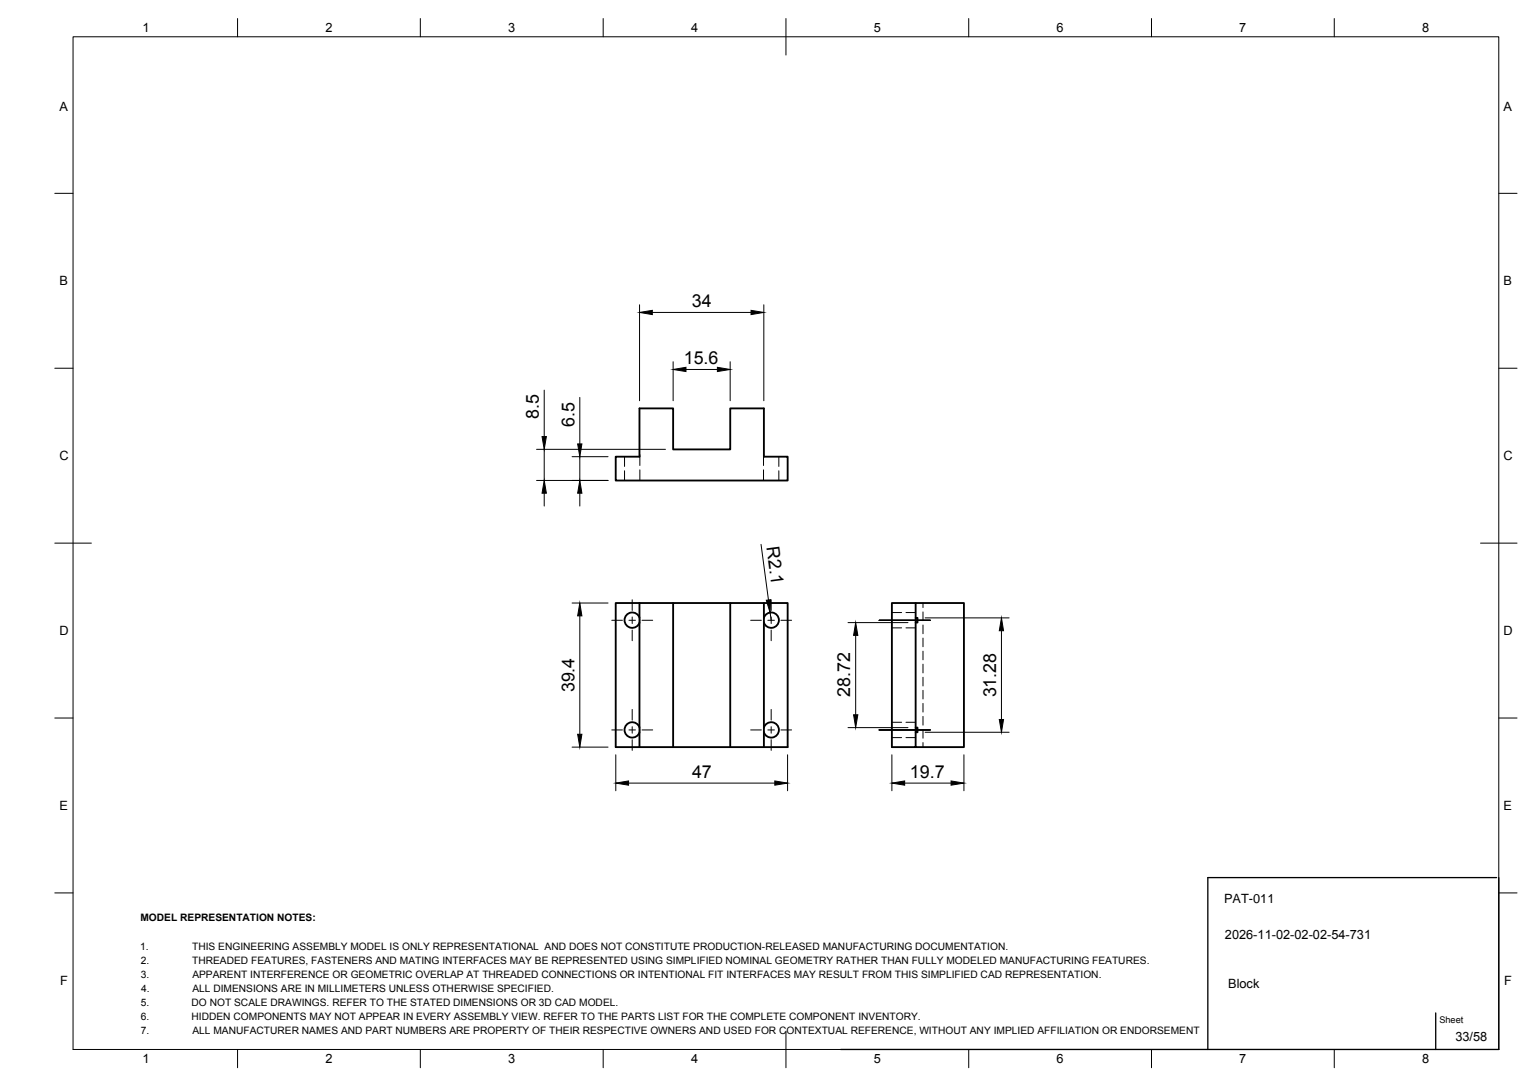
ISO-10303-21;
HEADER;
/* Generated by software containing ST-Developer
 * from STEP Tools, Inc. (www.steptools.com) 
 */

FILE_DESCRIPTION(
/* description */ ('Belt tension measurement rig'),
/* implementation_level */ '2;1');

FILE_NAME(
/* name */ 'Block.step',
/* time_stamp */ '2026-10-28T03:24:44-07:00',
/* author */ (''),
/* organization */ (''),
/* preprocessor_version */ 'ST-DEVELOPER v20.2',
/* originating_system */ 'Autodesk Translation Framework v15.17.0.0',
/* authorisation */ '');

FILE_SCHEMA (('AUTOMOTIVE_DESIGN { 1 0 10303 214 3 1 1 }'));
ENDSEC;

DATA;
#10=MECHANICAL_DESIGN_GEOMETRIC_PRESENTATION_REPRESENTATION('',(#727),#23587);
#609=SHAPE_REPRESENTATION_RELATIONSHIP('SRR','None',#23857,#664);
#664=ADVANCED_BREP_SHAPE_REPRESENTATION('',(#797),#23555);
#727=STYLED_ITEM('',(#24190),#797);
#797=MANIFOLD_SOLID_BREP('Body1',#12232);
#969=FACE_BOUND('',#2535,.T.);
#970=FACE_BOUND('',#2536,.T.);
#971=FACE_BOUND('',#2537,.T.);
#972=FACE_BOUND('',#2538,.T.);
#1201=PLANE('',#13566);
#1202=PLANE('',#13572);
#1203=PLANE('',#13578);
#1204=PLANE('',#13584);
#1205=PLANE('',#13590);
#1206=PLANE('',#13591);
#1207=PLANE('',#13592);
#1208=PLANE('',#13593);
#1209=PLANE('',#13594);
#1210=PLANE('',#13595);
#1211=PLANE('',#13596);
#1212=PLANE('',#13597);
#1213=PLANE('',#13598);
#1214=PLANE('',#13599);
#1215=PLANE('',#13600);
#1216=PLANE('',#13601);
#1217=PLANE('',#13602);
#1218=PLANE('',#13603);
#1677=FACE_OUTER_BOUND('',#2521,.T.);
#1678=FACE_OUTER_BOUND('',#2522,.T.);
#1679=FACE_OUTER_BOUND('',#2523,.T.);
#1680=FACE_OUTER_BOUND('',#2524,.T.);
#1681=FACE_OUTER_BOUND('',#2525,.T.);
#1682=FACE_OUTER_BOUND('',#2526,.T.);
#1683=FACE_OUTER_BOUND('',#2527,.T.);
#1684=FACE_OUTER_BOUND('',#2528,.T.);
#1685=FACE_OUTER_BOUND('',#2529,.T.);
#1686=FACE_OUTER_BOUND('',#2530,.T.);
#1687=FACE_OUTER_BOUND('',#2531,.T.);
#1688=FACE_OUTER_BOUND('',#2532,.T.);
#1689=FACE_OUTER_BOUND('',#2533,.T.);
#1690=FACE_OUTER_BOUND('',#2534,.T.);
#1691=FACE_OUTER_BOUND('',#2539,.T.);
#1692=FACE_OUTER_BOUND('',#2540,.T.);
#1693=FACE_OUTER_BOUND('',#2541,.T.);
#1694=FACE_OUTER_BOUND('',#2542,.T.);
#1695=FACE_OUTER_BOUND('',#2543,.T.);
#1696=FACE_OUTER_BOUND('',#2544,.T.);
#1697=FACE_OUTER_BOUND('',#2545,.T.);
#1698=FACE_OUTER_BOUND('',#2546,.T.);
#2521=EDGE_LOOP('',(#9362,#9363));
#2522=EDGE_LOOP('',(#9364,#9365,#9366,#9367,#9368,#9369,#9370,#9371));
#2523=EDGE_LOOP('',(#9372,#9373));
#2524=EDGE_LOOP('',(#9374,#9375,#9376,#9377,#9378,#9379,#9380,#9381));
#2525=EDGE_LOOP('',(#9382,#9383));
#2526=EDGE_LOOP('',(#9384,#9385,#9386,#9387,#9388,#9389,#9390,#9391));
#2527=EDGE_LOOP('',(#9392,#9393));
#2528=EDGE_LOOP('',(#9394,#9395,#9396,#9397,#9398,#9399,#9400,#9401));
#2529=EDGE_LOOP('',(#9402,#9403,#9404,#9405,#9406,#9407,#9408,#9409,#9410,
#9411,#9412,#9413));
#2530=EDGE_LOOP('',(#9414,#9415,#9416,#9417,#9418,#9419,#9420,#9421,#9422,
#9423,#9424,#9425));
#2531=EDGE_LOOP('',(#9426,#9427,#9428,#9429,#9430,#9431,#9432,#9433,#9434,
#9435,#9436,#9437));
#2532=EDGE_LOOP('',(#9438,#9439,#9440,#9441,#9442,#9443,#9444,#9445,#9446,
#9447));
#2533=EDGE_LOOP('',(#9448,#9449,#9450,#9451));
#2534=EDGE_LOOP('',(#9452,#9453,#9454,#9455));
#2535=EDGE_LOOP('',(#9456));
#2536=EDGE_LOOP('',(#9457));
#2537=EDGE_LOOP('',(#9458));
#2538=EDGE_LOOP('',(#9459));
#2539=EDGE_LOOP('',(#9460,#9461,#9462,#9463));
#2540=EDGE_LOOP('',(#9464,#9465,#9466,#9467,#9468,#9469,#9470,#9471,#9472,
#9473));
#2541=EDGE_LOOP('',(#9474,#9475,#9476,#9477));
#2542=EDGE_LOOP('',(#9478,#9479,#9480,#9481));
#2543=EDGE_LOOP('',(#9482,#9483,#9484,#9485));
#2544=EDGE_LOOP('',(#9486,#9487,#9488,#9489));
#2545=EDGE_LOOP('',(#9490,#9491,#9492,#9493));
#2546=EDGE_LOOP('',(#9494,#9495,#9496,#9497,#9498,#9499,#9500,#9501,#9502,
#9503,#9504,#9505));
#3327=LINE('',#20539,#4078);
#3328=LINE('',#20543,#4079);
#3329=LINE('',#20547,#4080);
#3330=LINE('',#20551,#4081);
#3331=LINE('',#20555,#4082);
#3332=LINE('',#20559,#4083);
#3333=LINE('',#20563,#4084);
#3334=LINE('',#20567,#4085);
#3335=LINE('',#20571,#4086);
#3336=LINE('',#20575,#4087);
#3337=LINE('',#20579,#4088);
#3338=LINE('',#20583,#4089);
#3339=LINE('',#20587,#4090);
#3340=LINE('',#20591,#4091);
#3341=LINE('',#20595,#4092);
#3342=LINE('',#20599,#4093);
#3343=LINE('',#20601,#4094);
#3344=LINE('',#20603,#4095);
#3345=LINE('',#20605,#4096);
#3346=LINE('',#20607,#4097);
#3347=LINE('',#20609,#4098);
#3348=LINE('',#20610,#4099);
#3349=LINE('',#20612,#4100);
#3350=LINE('',#20614,#4101);
#3351=LINE('',#20616,#4102);
#3352=LINE('',#20618,#4103);
#3353=LINE('',#20620,#4104);
#3354=LINE('',#20621,#4105);
#3355=LINE('',#20624,#4106);
#3356=LINE('',#20626,#4107);
#3357=LINE('',#20628,#4108);
#3358=LINE('',#20630,#4109);
#3359=LINE('',#20631,#4110);
#3360=LINE('',#20633,#4111);
#3361=LINE('',#20635,#4112);
#3362=LINE('',#20637,#4113);
#3363=LINE('',#20639,#4114);
#3364=LINE('',#20640,#4115);
#3365=LINE('',#20643,#4116);
#3366=LINE('',#20644,#4117);
#3367=LINE('',#20647,#4118);
#3368=LINE('',#20648,#4119);
#3369=LINE('',#20651,#4120);
#3370=LINE('',#20652,#4121);
#3371=LINE('',#20655,#4122);
#3372=LINE('',#20656,#4123);
#3373=LINE('',#20658,#4124);
#3374=LINE('',#20661,#4125);
#3375=LINE('',#20662,#4126);
#3376=LINE('',#20665,#4127);
#3377=LINE('',#20666,#4128);
#3378=LINE('',#20669,#4129);
#3379=LINE('',#20670,#4130);
#3380=LINE('',#20673,#4131);
#3381=LINE('',#20674,#4132);
#3382=LINE('',#20676,#4133);
#4078=VECTOR('',#16258,1.);
#4079=VECTOR('',#16263,1.);
#4080=VECTOR('',#16266,0.21);
#4081=VECTOR('',#16271,1.);
#4082=VECTOR('',#16274,1.);
#4083=VECTOR('',#16279,1.);
#4084=VECTOR('',#16282,0.21);
#4085=VECTOR('',#16287,1.);
#4086=VECTOR('',#16290,1.);
#4087=VECTOR('',#16295,1.);
#4088=VECTOR('',#16298,0.21);
#4089=VECTOR('',#16303,1.);
#4090=VECTOR('',#16306,1.);
#4091=VECTOR('',#16311,1.);
#4092=VECTOR('',#16314,0.21);
#4093=VECTOR('',#16319,1.);
#4094=VECTOR('',#16322,1.);
#4095=VECTOR('',#16323,1.);
#4096=VECTOR('',#16324,1.);
#4097=VECTOR('',#16325,1.);
#4098=VECTOR('',#16326,1.);
#4099=VECTOR('',#16327,1.);
#4100=VECTOR('',#16330,1.);
#4101=VECTOR('',#16331,1.);
#4102=VECTOR('',#16332,1.);
#4103=VECTOR('',#16333,1.);
#4104=VECTOR('',#16334,1.);
#4105=VECTOR('',#16335,1.);
#4106=VECTOR('',#16338,1.);
#4107=VECTOR('',#16339,1.);
#4108=VECTOR('',#16340,1.);
#4109=VECTOR('',#16341,1.);
#4110=VECTOR('',#16342,1.);
#4111=VECTOR('',#16343,1.);
#4112=VECTOR('',#16344,1.);
#4113=VECTOR('',#16345,1.);
#4114=VECTOR('',#16346,1.);
#4115=VECTOR('',#16347,1.);
#4116=VECTOR('',#16350,1.);
#4117=VECTOR('',#16351,1.);
#4118=VECTOR('',#16354,1.);
#4119=VECTOR('',#16355,1.);
#4120=VECTOR('',#16358,1.);
#4121=VECTOR('',#16359,1.);
#4122=VECTOR('',#16362,1.);
#4123=VECTOR('',#16363,1.);
#4124=VECTOR('',#16366,1.);
#4125=VECTOR('',#16369,1.);
#4126=VECTOR('',#16370,1.);
#4127=VECTOR('',#16373,1.);
#4128=VECTOR('',#16374,1.);
#4129=VECTOR('',#16377,1.);
#4130=VECTOR('',#16378,1.);
#4131=VECTOR('',#16381,1.);
#4132=VECTOR('',#16382,1.);
#4133=VECTOR('',#16385,1.);
#4797=CIRCLE('',#13567,0.21);
#4798=CIRCLE('',#13569,0.21);
#4799=CIRCLE('',#13570,0.21);
#4800=CIRCLE('',#13571,0.21);
#4801=CIRCLE('',#13573,0.21);
#4802=CIRCLE('',#13575,0.21);
#4803=CIRCLE('',#13576,0.21);
#4804=CIRCLE('',#13577,0.21);
#4805=CIRCLE('',#13579,0.21);
#4806=CIRCLE('',#13581,0.21);
#4807=CIRCLE('',#13582,0.21);
#4808=CIRCLE('',#13583,0.21);
#4809=CIRCLE('',#13585,0.21);
#4810=CIRCLE('',#13587,0.21);
#4811=CIRCLE('',#13588,0.21);
#4812=CIRCLE('',#13589,0.21);
#5719=VERTEX_POINT('',#20537);
#5720=VERTEX_POINT('',#20538);
#5721=VERTEX_POINT('',#20542);
#5722=VERTEX_POINT('',#20544);
#5723=VERTEX_POINT('',#20546);
#5724=VERTEX_POINT('',#20549);
#5725=VERTEX_POINT('',#20553);
#5726=VERTEX_POINT('',#20554);
#5727=VERTEX_POINT('',#20558);
#5728=VERTEX_POINT('',#20560);
#5729=VERTEX_POINT('',#20562);
#5730=VERTEX_POINT('',#20565);
#5731=VERTEX_POINT('',#20569);
#5732=VERTEX_POINT('',#20570);
#5733=VERTEX_POINT('',#20574);
#5734=VERTEX_POINT('',#20576);
#5735=VERTEX_POINT('',#20578);
#5736=VERTEX_POINT('',#20581);
#5737=VERTEX_POINT('',#20585);
#5738=VERTEX_POINT('',#20586);
#5739=VERTEX_POINT('',#20590);
#5740=VERTEX_POINT('',#20592);
#5741=VERTEX_POINT('',#20594);
#5742=VERTEX_POINT('',#20597);
#5743=VERTEX_POINT('',#20602);
#5744=VERTEX_POINT('',#20604);
#5745=VERTEX_POINT('',#20606);
#5746=VERTEX_POINT('',#20608);
#5747=VERTEX_POINT('',#20613);
#5748=VERTEX_POINT('',#20615);
#5749=VERTEX_POINT('',#20617);
#5750=VERTEX_POINT('',#20619);
#5751=VERTEX_POINT('',#20623);
#5752=VERTEX_POINT('',#20625);
#5753=VERTEX_POINT('',#20627);
#5754=VERTEX_POINT('',#20629);
#5755=VERTEX_POINT('',#20632);
#5756=VERTEX_POINT('',#20634);
#5757=VERTEX_POINT('',#20636);
#5758=VERTEX_POINT('',#20638);
#5759=VERTEX_POINT('',#20642);
#5760=VERTEX_POINT('',#20646);
#5761=VERTEX_POINT('',#20650);
#5762=VERTEX_POINT('',#20654);
#5763=VERTEX_POINT('',#20660);
#5764=VERTEX_POINT('',#20664);
#5765=VERTEX_POINT('',#20668);
#5766=VERTEX_POINT('',#20672);
#7040=EDGE_CURVE('',#5719,#5720,#3327,.T.);
#7041=EDGE_CURVE('',#5719,#5720,#4797,.T.);
#7042=EDGE_CURVE('',#5721,#5719,#3328,.T.);
#7043=EDGE_CURVE('',#5722,#5721,#4798,.T.);
#7044=EDGE_CURVE('',#5722,#5723,#3329,.T.);
#7045=EDGE_CURVE('',#5723,#5723,#4799,.T.);
#7046=EDGE_CURVE('',#5724,#5722,#4800,.T.);
#7047=EDGE_CURVE('',#5720,#5724,#3330,.T.);
#7048=EDGE_CURVE('',#5725,#5726,#3331,.T.);
#7049=EDGE_CURVE('',#5725,#5726,#4801,.T.);
#7050=EDGE_CURVE('',#5727,#5725,#3332,.T.);
#7051=EDGE_CURVE('',#5728,#5727,#4802,.T.);
#7052=EDGE_CURVE('',#5728,#5729,#3333,.T.);
#7053=EDGE_CURVE('',#5729,#5729,#4803,.T.);
#7054=EDGE_CURVE('',#5730,#5728,#4804,.T.);
#7055=EDGE_CURVE('',#5726,#5730,#3334,.T.);
#7056=EDGE_CURVE('',#5731,#5732,#3335,.T.);
#7057=EDGE_CURVE('',#5731,#5732,#4805,.T.);
#7058=EDGE_CURVE('',#5733,#5731,#3336,.T.);
#7059=EDGE_CURVE('',#5734,#5733,#4806,.T.);
#7060=EDGE_CURVE('',#5734,#5735,#3337,.T.);
#7061=EDGE_CURVE('',#5735,#5735,#4807,.T.);
#7062=EDGE_CURVE('',#5736,#5734,#4808,.T.);
#7063=EDGE_CURVE('',#5732,#5736,#3338,.T.);
#7064=EDGE_CURVE('',#5737,#5738,#3339,.T.);
#7065=EDGE_CURVE('',#5737,#5738,#4809,.T.);
#7066=EDGE_CURVE('',#5739,#5737,#3340,.T.);
#7067=EDGE_CURVE('',#5740,#5739,#4810,.T.);
#7068=EDGE_CURVE('',#5740,#5741,#3341,.T.);
#7069=EDGE_CURVE('',#5741,#5741,#4811,.T.);
#7070=EDGE_CURVE('',#5742,#5740,#4812,.T.);
#7071=EDGE_CURVE('',#5738,#5742,#3342,.T.);
#7072=EDGE_CURVE('',#5724,#5733,#3343,.T.);
#7073=EDGE_CURVE('',#5736,#5743,#3344,.T.);
#7074=EDGE_CURVE('',#5744,#5743,#3345,.T.);
#7075=EDGE_CURVE('',#5744,#5745,#3346,.T.);
#7076=EDGE_CURVE('',#5746,#5745,#3347,.T.);
#7077=EDGE_CURVE('',#5746,#5721,#3348,.T.);
#7078=EDGE_CURVE('',#5730,#5739,#3349,.T.);
#7079=EDGE_CURVE('',#5742,#5747,#3350,.T.);
#7080=EDGE_CURVE('',#5748,#5747,#3351,.T.);
#7081=EDGE_CURVE('',#5749,#5748,#3352,.T.);
#7082=EDGE_CURVE('',#5750,#5749,#3353,.T.);
#7083=EDGE_CURVE('',#5750,#5727,#3354,.T.);
#7084=EDGE_CURVE('',#5743,#5751,#3355,.T.);
#7085=EDGE_CURVE('',#5751,#5752,#3356,.T.);
#7086=EDGE_CURVE('',#5752,#5753,#3357,.T.);
#7087=EDGE_CURVE('',#5753,#5754,#3358,.T.);
#7088=EDGE_CURVE('',#5754,#5750,#3359,.T.);
#7089=EDGE_CURVE('',#5749,#5755,#3360,.T.);
#7090=EDGE_CURVE('',#5755,#5756,#3361,.T.);
#7091=EDGE_CURVE('',#5756,#5757,#3362,.T.);
#7092=EDGE_CURVE('',#5757,#5758,#3363,.T.);
#7093=EDGE_CURVE('',#5758,#5744,#3364,.T.);
#7094=EDGE_CURVE('',#5759,#5746,#3365,.T.);
#7095=EDGE_CURVE('',#5751,#5759,#3366,.T.);
#7096=EDGE_CURVE('',#5760,#5759,#3367,.T.);
#7097=EDGE_CURVE('',#5752,#5760,#3368,.T.);
#7098=EDGE_CURVE('',#5761,#5760,#3369,.T.);
#7099=EDGE_CURVE('',#5753,#5761,#3370,.T.);
#7100=EDGE_CURVE('',#5762,#5761,#3371,.T.);
#7101=EDGE_CURVE('',#5754,#5762,#3372,.T.);
#7102=EDGE_CURVE('',#5747,#5762,#3373,.T.);
#7103=EDGE_CURVE('',#5763,#5748,#3374,.T.);
#7104=EDGE_CURVE('',#5755,#5763,#3375,.T.);
#7105=EDGE_CURVE('',#5764,#5763,#3376,.T.);
#7106=EDGE_CURVE('',#5756,#5764,#3377,.T.);
#7107=EDGE_CURVE('',#5765,#5764,#3378,.T.);
#7108=EDGE_CURVE('',#5757,#5765,#3379,.T.);
#7109=EDGE_CURVE('',#5766,#5765,#3380,.T.);
#7110=EDGE_CURVE('',#5758,#5766,#3381,.T.);
#7111=EDGE_CURVE('',#5745,#5766,#3382,.T.);
#9362=ORIENTED_EDGE('',*,*,#7040,.F.);
#9363=ORIENTED_EDGE('',*,*,#7041,.T.);
#9364=ORIENTED_EDGE('',*,*,#7042,.F.);
#9365=ORIENTED_EDGE('',*,*,#7043,.F.);
#9366=ORIENTED_EDGE('',*,*,#7044,.T.);
#9367=ORIENTED_EDGE('',*,*,#7045,.F.);
#9368=ORIENTED_EDGE('',*,*,#7044,.F.);
#9369=ORIENTED_EDGE('',*,*,#7046,.F.);
#9370=ORIENTED_EDGE('',*,*,#7047,.F.);
#9371=ORIENTED_EDGE('',*,*,#7041,.F.);
#9372=ORIENTED_EDGE('',*,*,#7048,.F.);
#9373=ORIENTED_EDGE('',*,*,#7049,.T.);
#9374=ORIENTED_EDGE('',*,*,#7050,.F.);
#9375=ORIENTED_EDGE('',*,*,#7051,.F.);
#9376=ORIENTED_EDGE('',*,*,#7052,.T.);
#9377=ORIENTED_EDGE('',*,*,#7053,.F.);
#9378=ORIENTED_EDGE('',*,*,#7052,.F.);
#9379=ORIENTED_EDGE('',*,*,#7054,.F.);
#9380=ORIENTED_EDGE('',*,*,#7055,.F.);
#9381=ORIENTED_EDGE('',*,*,#7049,.F.);
#9382=ORIENTED_EDGE('',*,*,#7056,.F.);
#9383=ORIENTED_EDGE('',*,*,#7057,.T.);
#9384=ORIENTED_EDGE('',*,*,#7058,.F.);
#9385=ORIENTED_EDGE('',*,*,#7059,.F.);
#9386=ORIENTED_EDGE('',*,*,#7060,.T.);
#9387=ORIENTED_EDGE('',*,*,#7061,.F.);
#9388=ORIENTED_EDGE('',*,*,#7060,.F.);
#9389=ORIENTED_EDGE('',*,*,#7062,.F.);
#9390=ORIENTED_EDGE('',*,*,#7063,.F.);
#9391=ORIENTED_EDGE('',*,*,#7057,.F.);
#9392=ORIENTED_EDGE('',*,*,#7064,.F.);
#9393=ORIENTED_EDGE('',*,*,#7065,.T.);
#9394=ORIENTED_EDGE('',*,*,#7066,.F.);
#9395=ORIENTED_EDGE('',*,*,#7067,.F.);
#9396=ORIENTED_EDGE('',*,*,#7068,.T.);
#9397=ORIENTED_EDGE('',*,*,#7069,.F.);
#9398=ORIENTED_EDGE('',*,*,#7068,.F.);
#9399=ORIENTED_EDGE('',*,*,#7070,.F.);
#9400=ORIENTED_EDGE('',*,*,#7071,.F.);
#9401=ORIENTED_EDGE('',*,*,#7065,.F.);
#9402=ORIENTED_EDGE('',*,*,#7042,.T.);
#9403=ORIENTED_EDGE('',*,*,#7040,.T.);
#9404=ORIENTED_EDGE('',*,*,#7047,.T.);
#9405=ORIENTED_EDGE('',*,*,#7072,.T.);
#9406=ORIENTED_EDGE('',*,*,#7058,.T.);
#9407=ORIENTED_EDGE('',*,*,#7056,.T.);
#9408=ORIENTED_EDGE('',*,*,#7063,.T.);
#9409=ORIENTED_EDGE('',*,*,#7073,.T.);
#9410=ORIENTED_EDGE('',*,*,#7074,.F.);
#9411=ORIENTED_EDGE('',*,*,#7075,.T.);
#9412=ORIENTED_EDGE('',*,*,#7076,.F.);
#9413=ORIENTED_EDGE('',*,*,#7077,.T.);
#9414=ORIENTED_EDGE('',*,*,#7050,.T.);
#9415=ORIENTED_EDGE('',*,*,#7048,.T.);
#9416=ORIENTED_EDGE('',*,*,#7055,.T.);
#9417=ORIENTED_EDGE('',*,*,#7078,.T.);
#9418=ORIENTED_EDGE('',*,*,#7066,.T.);
#9419=ORIENTED_EDGE('',*,*,#7064,.T.);
#9420=ORIENTED_EDGE('',*,*,#7071,.T.);
#9421=ORIENTED_EDGE('',*,*,#7079,.T.);
#9422=ORIENTED_EDGE('',*,*,#7080,.F.);
#9423=ORIENTED_EDGE('',*,*,#7081,.F.);
#9424=ORIENTED_EDGE('',*,*,#7082,.F.);
#9425=ORIENTED_EDGE('',*,*,#7083,.T.);
#9426=ORIENTED_EDGE('',*,*,#7074,.T.);
#9427=ORIENTED_EDGE('',*,*,#7084,.T.);
#9428=ORIENTED_EDGE('',*,*,#7085,.T.);
#9429=ORIENTED_EDGE('',*,*,#7086,.T.);
#9430=ORIENTED_EDGE('',*,*,#7087,.T.);
#9431=ORIENTED_EDGE('',*,*,#7088,.T.);
#9432=ORIENTED_EDGE('',*,*,#7082,.T.);
#9433=ORIENTED_EDGE('',*,*,#7089,.T.);
#9434=ORIENTED_EDGE('',*,*,#7090,.T.);
#9435=ORIENTED_EDGE('',*,*,#7091,.T.);
#9436=ORIENTED_EDGE('',*,*,#7092,.T.);
#9437=ORIENTED_EDGE('',*,*,#7093,.T.);
#9438=ORIENTED_EDGE('',*,*,#7046,.T.);
#9439=ORIENTED_EDGE('',*,*,#7043,.T.);
#9440=ORIENTED_EDGE('',*,*,#7077,.F.);
#9441=ORIENTED_EDGE('',*,*,#7094,.F.);
#9442=ORIENTED_EDGE('',*,*,#7095,.F.);
#9443=ORIENTED_EDGE('',*,*,#7084,.F.);
#9444=ORIENTED_EDGE('',*,*,#7073,.F.);
#9445=ORIENTED_EDGE('',*,*,#7062,.T.);
#9446=ORIENTED_EDGE('',*,*,#7059,.T.);
#9447=ORIENTED_EDGE('',*,*,#7072,.F.);
#9448=ORIENTED_EDGE('',*,*,#7095,.T.);
#9449=ORIENTED_EDGE('',*,*,#7096,.F.);
#9450=ORIENTED_EDGE('',*,*,#7097,.F.);
#9451=ORIENTED_EDGE('',*,*,#7085,.F.);
#9452=ORIENTED_EDGE('',*,*,#7097,.T.);
#9453=ORIENTED_EDGE('',*,*,#7098,.F.);
#9454=ORIENTED_EDGE('',*,*,#7099,.F.);
#9455=ORIENTED_EDGE('',*,*,#7086,.F.);
#9456=ORIENTED_EDGE('',*,*,#7045,.T.);
#9457=ORIENTED_EDGE('',*,*,#7053,.T.);
#9458=ORIENTED_EDGE('',*,*,#7061,.T.);
#9459=ORIENTED_EDGE('',*,*,#7069,.T.);
#9460=ORIENTED_EDGE('',*,*,#7099,.T.);
#9461=ORIENTED_EDGE('',*,*,#7100,.F.);
#9462=ORIENTED_EDGE('',*,*,#7101,.F.);
#9463=ORIENTED_EDGE('',*,*,#7087,.F.);
#9464=ORIENTED_EDGE('',*,*,#7054,.T.);
#9465=ORIENTED_EDGE('',*,*,#7051,.T.);
#9466=ORIENTED_EDGE('',*,*,#7083,.F.);
#9467=ORIENTED_EDGE('',*,*,#7088,.F.);
#9468=ORIENTED_EDGE('',*,*,#7101,.T.);
#9469=ORIENTED_EDGE('',*,*,#7102,.F.);
#9470=ORIENTED_EDGE('',*,*,#7079,.F.);
#9471=ORIENTED_EDGE('',*,*,#7070,.T.);
#9472=ORIENTED_EDGE('',*,*,#7067,.T.);
#9473=ORIENTED_EDGE('',*,*,#7078,.F.);
#9474=ORIENTED_EDGE('',*,*,#7081,.T.);
#9475=ORIENTED_EDGE('',*,*,#7103,.F.);
#9476=ORIENTED_EDGE('',*,*,#7104,.F.);
#9477=ORIENTED_EDGE('',*,*,#7089,.F.);
#9478=ORIENTED_EDGE('',*,*,#7104,.T.);
#9479=ORIENTED_EDGE('',*,*,#7105,.F.);
#9480=ORIENTED_EDGE('',*,*,#7106,.F.);
#9481=ORIENTED_EDGE('',*,*,#7090,.F.);
#9482=ORIENTED_EDGE('',*,*,#7106,.T.);
#9483=ORIENTED_EDGE('',*,*,#7107,.F.);
#9484=ORIENTED_EDGE('',*,*,#7108,.F.);
#9485=ORIENTED_EDGE('',*,*,#7091,.F.);
#9486=ORIENTED_EDGE('',*,*,#7108,.T.);
#9487=ORIENTED_EDGE('',*,*,#7109,.F.);
#9488=ORIENTED_EDGE('',*,*,#7110,.F.);
#9489=ORIENTED_EDGE('',*,*,#7092,.F.);
#9490=ORIENTED_EDGE('',*,*,#7110,.T.);
#9491=ORIENTED_EDGE('',*,*,#7111,.F.);
#9492=ORIENTED_EDGE('',*,*,#7075,.F.);
#9493=ORIENTED_EDGE('',*,*,#7093,.F.);
#9494=ORIENTED_EDGE('',*,*,#7076,.T.);
#9495=ORIENTED_EDGE('',*,*,#7111,.T.);
#9496=ORIENTED_EDGE('',*,*,#7109,.T.);
#9497=ORIENTED_EDGE('',*,*,#7107,.T.);
#9498=ORIENTED_EDGE('',*,*,#7105,.T.);
#9499=ORIENTED_EDGE('',*,*,#7103,.T.);
#9500=ORIENTED_EDGE('',*,*,#7080,.T.);
#9501=ORIENTED_EDGE('',*,*,#7102,.T.);
#9502=ORIENTED_EDGE('',*,*,#7100,.T.);
#9503=ORIENTED_EDGE('',*,*,#7098,.T.);
#9504=ORIENTED_EDGE('',*,*,#7096,.T.);
#9505=ORIENTED_EDGE('',*,*,#7094,.T.);
#11297=CYLINDRICAL_SURFACE('',#13568,0.21);
#11298=CYLINDRICAL_SURFACE('',#13574,0.21);
#11299=CYLINDRICAL_SURFACE('',#13580,0.21);
#11300=CYLINDRICAL_SURFACE('',#13586,0.21);
#11818=ADVANCED_FACE('',(#1677),#1201,.T.);
#11819=ADVANCED_FACE('',(#1678),#11297,.F.);
#11820=ADVANCED_FACE('',(#1679),#1202,.T.);
#11821=ADVANCED_FACE('',(#1680),#11298,.F.);
#11822=ADVANCED_FACE('',(#1681),#1203,.T.);
#11823=ADVANCED_FACE('',(#1682),#11299,.F.);
#11824=ADVANCED_FACE('',(#1683),#1204,.T.);
#11825=ADVANCED_FACE('',(#1684),#11300,.F.);
#11826=ADVANCED_FACE('',(#1685),#1205,.T.);
#11827=ADVANCED_FACE('',(#1686),#1206,.T.);
#11828=ADVANCED_FACE('',(#1687),#1207,.T.);
#11829=ADVANCED_FACE('',(#1688),#1208,.T.);
#11830=ADVANCED_FACE('',(#1689),#1209,.T.);
#11831=ADVANCED_FACE('',(#1690,#969,#970,#971,#972),#1210,.T.);
#11832=ADVANCED_FACE('',(#1691),#1211,.T.);
#11833=ADVANCED_FACE('',(#1692),#1212,.T.);
#11834=ADVANCED_FACE('',(#1693),#1213,.T.);
#11835=ADVANCED_FACE('',(#1694),#1214,.T.);
#11836=ADVANCED_FACE('',(#1695),#1215,.T.);
#11837=ADVANCED_FACE('',(#1696),#1216,.T.);
#11838=ADVANCED_FACE('',(#1697),#1217,.T.);
#11839=ADVANCED_FACE('',(#1698),#1218,.T.);
#12232=CLOSED_SHELL('',(#11818,#11819,#11820,#11821,#11822,#11823,#11824,
#11825,#11826,#11827,#11828,#11829,#11830,#11831,#11832,#11833,#11834,#11835,
#11836,#11837,#11838,#11839));
#13565=AXIS2_PLACEMENT_3D('',#20535,#16254,#16255);
#13566=AXIS2_PLACEMENT_3D('',#20536,#16256,#16257);
#13567=AXIS2_PLACEMENT_3D('',#20540,#16259,#16260);
#13568=AXIS2_PLACEMENT_3D('',#20541,#16261,#16262);
#13569=AXIS2_PLACEMENT_3D('',#20545,#16264,#16265);
#13570=AXIS2_PLACEMENT_3D('',#20548,#16267,#16268);
#13571=AXIS2_PLACEMENT_3D('',#20550,#16269,#16270);
#13572=AXIS2_PLACEMENT_3D('',#20552,#16272,#16273);
#13573=AXIS2_PLACEMENT_3D('',#20556,#16275,#16276);
#13574=AXIS2_PLACEMENT_3D('',#20557,#16277,#16278);
#13575=AXIS2_PLACEMENT_3D('',#20561,#16280,#16281);
#13576=AXIS2_PLACEMENT_3D('',#20564,#16283,#16284);
#13577=AXIS2_PLACEMENT_3D('',#20566,#16285,#16286);
#13578=AXIS2_PLACEMENT_3D('',#20568,#16288,#16289);
#13579=AXIS2_PLACEMENT_3D('',#20572,#16291,#16292);
#13580=AXIS2_PLACEMENT_3D('',#20573,#16293,#16294);
#13581=AXIS2_PLACEMENT_3D('',#20577,#16296,#16297);
#13582=AXIS2_PLACEMENT_3D('',#20580,#16299,#16300);
#13583=AXIS2_PLACEMENT_3D('',#20582,#16301,#16302);
#13584=AXIS2_PLACEMENT_3D('',#20584,#16304,#16305);
#13585=AXIS2_PLACEMENT_3D('',#20588,#16307,#16308);
#13586=AXIS2_PLACEMENT_3D('',#20589,#16309,#16310);
#13587=AXIS2_PLACEMENT_3D('',#20593,#16312,#16313);
#13588=AXIS2_PLACEMENT_3D('',#20596,#16315,#16316);
#13589=AXIS2_PLACEMENT_3D('',#20598,#16317,#16318);
#13590=AXIS2_PLACEMENT_3D('',#20600,#16320,#16321);
#13591=AXIS2_PLACEMENT_3D('',#20611,#16328,#16329);
#13592=AXIS2_PLACEMENT_3D('',#20622,#16336,#16337);
#13593=AXIS2_PLACEMENT_3D('',#20641,#16348,#16349);
#13594=AXIS2_PLACEMENT_3D('',#20645,#16352,#16353);
#13595=AXIS2_PLACEMENT_3D('',#20649,#16356,#16357);
#13596=AXIS2_PLACEMENT_3D('',#20653,#16360,#16361);
#13597=AXIS2_PLACEMENT_3D('',#20657,#16364,#16365);
#13598=AXIS2_PLACEMENT_3D('',#20659,#16367,#16368);
#13599=AXIS2_PLACEMENT_3D('',#20663,#16371,#16372);
#13600=AXIS2_PLACEMENT_3D('',#20667,#16375,#16376);
#13601=AXIS2_PLACEMENT_3D('',#20671,#16379,#16380);
#13602=AXIS2_PLACEMENT_3D('',#20675,#16383,#16384);
#13603=AXIS2_PLACEMENT_3D('',#20677,#16386,#16387);
#16254=DIRECTION('axis',(0.,0.,1.));
#16255=DIRECTION('refdir',(1.,0.,0.));
#16256=DIRECTION('center_axis',(0.,0.,1.));
#16257=DIRECTION('ref_axis',(1.,0.,0.));
#16258=DIRECTION('',(-1.,0.,0.));
#16259=DIRECTION('center_axis',(0.,0.,1.));
#16260=DIRECTION('ref_axis',(1.,0.,0.));
#16261=DIRECTION('center_axis',(0.,0.,1.));
#16262=DIRECTION('ref_axis',(1.,0.,0.));
#16263=DIRECTION('',(0.,0.,-1.));
#16264=DIRECTION('center_axis',(0.,0.,1.));
#16265=DIRECTION('ref_axis',(1.,0.,0.));
#16266=DIRECTION('',(0.,0.,1.));
#16267=DIRECTION('center_axis',(0.,0.,-1.));
#16268=DIRECTION('ref_axis',(1.,0.,0.));
#16269=DIRECTION('center_axis',(0.,0.,1.));
#16270=DIRECTION('ref_axis',(1.,0.,0.));
#16271=DIRECTION('',(0.,0.,1.));
#16272=DIRECTION('center_axis',(0.,0.,1.));
#16273=DIRECTION('ref_axis',(1.,0.,0.));
#16274=DIRECTION('',(1.,0.,0.));
#16275=DIRECTION('center_axis',(0.,0.,1.));
#16276=DIRECTION('ref_axis',(1.,0.,0.));
#16277=DIRECTION('center_axis',(0.,0.,1.));
#16278=DIRECTION('ref_axis',(1.,0.,0.));
#16279=DIRECTION('',(0.,0.,-1.));
#16280=DIRECTION('center_axis',(0.,0.,1.));
#16281=DIRECTION('ref_axis',(1.,0.,0.));
#16282=DIRECTION('',(0.,0.,1.));
#16283=DIRECTION('center_axis',(0.,0.,-1.));
#16284=DIRECTION('ref_axis',(1.,0.,0.));
#16285=DIRECTION('center_axis',(0.,0.,1.));
#16286=DIRECTION('ref_axis',(1.,0.,0.));
#16287=DIRECTION('',(0.,0.,1.));
#16288=DIRECTION('center_axis',(0.,0.,1.));
#16289=DIRECTION('ref_axis',(1.,0.,0.));
#16290=DIRECTION('',(-1.,0.,0.));
#16291=DIRECTION('center_axis',(0.,0.,1.));
#16292=DIRECTION('ref_axis',(1.,0.,0.));
#16293=DIRECTION('center_axis',(0.,0.,1.));
#16294=DIRECTION('ref_axis',(1.,0.,0.));
#16295=DIRECTION('',(0.,0.,-1.));
#16296=DIRECTION('center_axis',(0.,0.,1.));
#16297=DIRECTION('ref_axis',(1.,0.,0.));
#16298=DIRECTION('',(0.,0.,1.));
#16299=DIRECTION('center_axis',(0.,0.,-1.));
#16300=DIRECTION('ref_axis',(1.,0.,0.));
#16301=DIRECTION('center_axis',(0.,0.,1.));
#16302=DIRECTION('ref_axis',(1.,0.,0.));
#16303=DIRECTION('',(0.,0.,1.));
#16304=DIRECTION('center_axis',(0.,0.,1.));
#16305=DIRECTION('ref_axis',(1.,0.,0.));
#16306=DIRECTION('',(1.,0.,0.));
#16307=DIRECTION('center_axis',(0.,0.,1.));
#16308=DIRECTION('ref_axis',(1.,0.,0.));
#16309=DIRECTION('center_axis',(0.,0.,1.));
#16310=DIRECTION('ref_axis',(1.,0.,0.));
#16311=DIRECTION('',(0.,0.,-1.));
#16312=DIRECTION('center_axis',(0.,0.,1.));
#16313=DIRECTION('ref_axis',(1.,0.,0.));
#16314=DIRECTION('',(0.,0.,1.));
#16315=DIRECTION('center_axis',(0.,0.,-1.));
#16316=DIRECTION('ref_axis',(1.,0.,0.));
#16317=DIRECTION('center_axis',(0.,0.,1.));
#16318=DIRECTION('ref_axis',(1.,0.,0.));
#16319=DIRECTION('',(0.,0.,1.));
#16320=DIRECTION('center_axis',(0.,-1.,0.));
#16321=DIRECTION('ref_axis',(0.,0.,-1.));
#16322=DIRECTION('',(-1.,0.,0.));
#16323=DIRECTION('',(-1.,0.,0.));
#16324=DIRECTION('',(0.,0.,1.));
#16325=DIRECTION('',(1.,0.,0.));
#16326=DIRECTION('',(0.,0.,-1.));
#16327=DIRECTION('',(-1.,0.,0.));
#16328=DIRECTION('center_axis',(0.,1.,0.));
#16329=DIRECTION('ref_axis',(0.,0.,1.));
#16330=DIRECTION('',(1.,0.,0.));
#16331=DIRECTION('',(1.,0.,0.));
#16332=DIRECTION('',(0.,0.,1.));
#16333=DIRECTION('',(1.,0.,0.));
#16334=DIRECTION('',(0.,0.,-1.));
#16335=DIRECTION('',(1.,0.,0.));
#16336=DIRECTION('center_axis',(-1.,0.,0.));
#16337=DIRECTION('ref_axis',(0.,0.,1.));
#16338=DIRECTION('',(0.,-1.,0.));
#16339=DIRECTION('',(0.,0.,1.));
#16340=DIRECTION('',(0.,1.,0.));
#16341=DIRECTION('',(0.,0.,-1.));
#16342=DIRECTION('',(0.,-1.,0.));
#16343=DIRECTION('',(0.,-1.,0.));
#16344=DIRECTION('',(0.,0.,1.));
#16345=DIRECTION('',(0.,-1.,0.));
#16346=DIRECTION('',(0.,0.,-1.));
#16347=DIRECTION('',(0.,-1.,0.));
#16348=DIRECTION('center_axis',(0.,0.,-1.));
#16349=DIRECTION('ref_axis',(0.,1.,0.));
#16350=DIRECTION('',(0.,1.,0.));
#16351=DIRECTION('',(1.,0.,0.));
#16352=DIRECTION('center_axis',(0.,-1.,0.));
#16353=DIRECTION('ref_axis',(0.,0.,-1.));
#16354=DIRECTION('',(0.,0.,-1.));
#16355=DIRECTION('',(1.,0.,0.));
#16356=DIRECTION('center_axis',(0.,0.,1.));
#16357=DIRECTION('ref_axis',(0.,-1.,0.));
#16358=DIRECTION('',(0.,-1.,0.));
#16359=DIRECTION('',(1.,0.,0.));
#16360=DIRECTION('center_axis',(0.,1.,0.));
#16361=DIRECTION('ref_axis',(0.,0.,1.));
#16362=DIRECTION('',(0.,0.,1.));
#16363=DIRECTION('',(1.,0.,0.));
#16364=DIRECTION('center_axis',(0.,0.,-1.));
#16365=DIRECTION('ref_axis',(0.,1.,0.));
#16366=DIRECTION('',(0.,1.,0.));
#16367=DIRECTION('center_axis',(0.,0.,-1.));
#16368=DIRECTION('ref_axis',(0.,1.,0.));
#16369=DIRECTION('',(0.,1.,0.));
#16370=DIRECTION('',(1.,0.,0.));
#16371=DIRECTION('center_axis',(0.,-1.,0.));
#16372=DIRECTION('ref_axis',(0.,0.,-1.));
#16373=DIRECTION('',(0.,0.,-1.));
#16374=DIRECTION('',(1.,0.,0.));
#16375=DIRECTION('center_axis',(0.,0.,-1.));
#16376=DIRECTION('ref_axis',(0.,1.,0.));
#16377=DIRECTION('',(0.,1.,0.));
#16378=DIRECTION('',(1.,0.,0.));
#16379=DIRECTION('center_axis',(0.,1.,0.));
#16380=DIRECTION('ref_axis',(0.,0.,1.));
#16381=DIRECTION('',(0.,0.,1.));
#16382=DIRECTION('',(1.,0.,0.));
#16383=DIRECTION('center_axis',(0.,0.,-1.));
#16384=DIRECTION('ref_axis',(0.,1.,0.));
#16385=DIRECTION('',(0.,1.,0.));
#16386=DIRECTION('center_axis',(1.,0.,0.));
#16387=DIRECTION('ref_axis',(0.,0.,-1.));
#20535=CARTESIAN_POINT('',(0.,0.,0.));
#20536=CARTESIAN_POINT('Origin',(1.5,-1.9,1.7));
#20537=CARTESIAN_POINT('',(1.56403124237433,-1.7,1.7));
#20538=CARTESIAN_POINT('',(1.43596875762567,-1.7,1.7));
#20539=CARTESIAN_POINT('',(0.75,-1.7,1.7));
#20540=CARTESIAN_POINT('Origin',(1.5,-1.9,1.7));
#20541=CARTESIAN_POINT('Origin',(1.5,-1.9,1.7));
#20542=CARTESIAN_POINT('',(1.56403124237433,-1.7,1.75));
#20543=CARTESIAN_POINT('',(1.56403124237433,-1.7,1.7));
#20544=CARTESIAN_POINT('',(1.29,-1.9,1.75));
#20545=CARTESIAN_POINT('Origin',(1.5,-1.9,1.75));
#20546=CARTESIAN_POINT('',(1.29,-1.9,2.4));
#20547=CARTESIAN_POINT('',(1.29,-1.9,1.7));
#20548=CARTESIAN_POINT('Origin',(1.5,-1.9,2.4));
#20549=CARTESIAN_POINT('',(1.43596875762567,-1.7,1.75));
#20550=CARTESIAN_POINT('Origin',(1.5,-1.9,1.75));
#20551=CARTESIAN_POINT('',(1.43596875762567,-1.7,1.7));
#20552=CARTESIAN_POINT('Origin',(-1.5,1.9,1.7));
#20553=CARTESIAN_POINT('',(-1.56403124237433,1.7,1.7));
#20554=CARTESIAN_POINT('',(-1.43596875762567,1.7,1.7));
#20555=CARTESIAN_POINT('',(-0.75,1.7,1.7));
#20556=CARTESIAN_POINT('Origin',(-1.5,1.9,1.7));
#20557=CARTESIAN_POINT('Origin',(-1.5,1.9,1.7));
#20558=CARTESIAN_POINT('',(-1.56403124237433,1.7,1.75));
#20559=CARTESIAN_POINT('',(-1.56403124237433,1.7,1.7));
#20560=CARTESIAN_POINT('',(-1.71,1.9,1.75));
#20561=CARTESIAN_POINT('Origin',(-1.5,1.9,1.75));
#20562=CARTESIAN_POINT('',(-1.71,1.9,2.4));
#20563=CARTESIAN_POINT('',(-1.71,1.9,1.7));
#20564=CARTESIAN_POINT('Origin',(-1.5,1.9,2.4));
#20565=CARTESIAN_POINT('',(-1.43596875762567,1.7,1.75));
#20566=CARTESIAN_POINT('Origin',(-1.5,1.9,1.75));
#20567=CARTESIAN_POINT('',(-1.43596875762567,1.7,1.7));
#20568=CARTESIAN_POINT('Origin',(-1.5,-1.9,1.7));
#20569=CARTESIAN_POINT('',(-1.43596875762567,-1.7,1.7));
#20570=CARTESIAN_POINT('',(-1.56403124237433,-1.7,1.7));
#20571=CARTESIAN_POINT('',(-0.75,-1.7,1.7));
#20572=CARTESIAN_POINT('Origin',(-1.5,-1.9,1.7));
#20573=CARTESIAN_POINT('Origin',(-1.5,-1.9,1.7));
#20574=CARTESIAN_POINT('',(-1.43596875762567,-1.7,1.75));
#20575=CARTESIAN_POINT('',(-1.43596875762567,-1.7,1.7));
#20576=CARTESIAN_POINT('',(-1.71,-1.9,1.75));
#20577=CARTESIAN_POINT('Origin',(-1.5,-1.9,1.75));
#20578=CARTESIAN_POINT('',(-1.71,-1.9,2.4));
#20579=CARTESIAN_POINT('',(-1.71,-1.9,1.7));
#20580=CARTESIAN_POINT('Origin',(-1.5,-1.9,2.4));
#20581=CARTESIAN_POINT('',(-1.56403124237433,-1.7,1.75));
#20582=CARTESIAN_POINT('Origin',(-1.5,-1.9,1.75));
#20583=CARTESIAN_POINT('',(-1.56403124237433,-1.7,1.7));
#20584=CARTESIAN_POINT('Origin',(1.5,1.9,1.7));
#20585=CARTESIAN_POINT('',(1.43596875762567,1.7,1.7));
#20586=CARTESIAN_POINT('',(1.56403124237433,1.7,1.7));
#20587=CARTESIAN_POINT('',(0.75,1.7,1.7));
#20588=CARTESIAN_POINT('Origin',(1.5,1.9,1.7));
#20589=CARTESIAN_POINT('Origin',(1.5,1.9,1.7));
#20590=CARTESIAN_POINT('',(1.43596875762567,1.7,1.75));
#20591=CARTESIAN_POINT('',(1.43596875762567,1.7,1.7));
#20592=CARTESIAN_POINT('',(1.29,1.9,1.75));
#20593=CARTESIAN_POINT('Origin',(1.5,1.9,1.75));
#20594=CARTESIAN_POINT('',(1.29,1.9,2.4));
#20595=CARTESIAN_POINT('',(1.29,1.9,1.7));
#20596=CARTESIAN_POINT('Origin',(1.5,1.9,2.4));
#20597=CARTESIAN_POINT('',(1.56403124237433,1.7,1.75));
#20598=CARTESIAN_POINT('Origin',(1.5,1.9,1.75));
#20599=CARTESIAN_POINT('',(1.56403124237433,1.7,1.7));
#20600=CARTESIAN_POINT('Origin',(0.,-1.7,1.75));
#20601=CARTESIAN_POINT('',(0.,-1.7,1.75));
#20602=CARTESIAN_POINT('',(-1.97,-1.7,1.75));
#20603=CARTESIAN_POINT('',(0.,-1.7,1.75));
#20604=CARTESIAN_POINT('',(-1.97,-1.7,0.43));
#20605=CARTESIAN_POINT('',(-1.97,-1.7,1.75));
#20606=CARTESIAN_POINT('',(1.97,-1.7,0.43));
#20607=CARTESIAN_POINT('',(0.,-1.7,0.43));
#20608=CARTESIAN_POINT('',(1.97,-1.7,1.75));
#20609=CARTESIAN_POINT('',(1.97,-1.7,1.75));
#20610=CARTESIAN_POINT('',(0.,-1.7,1.75));
#20611=CARTESIAN_POINT('Origin',(0.,1.7,0.43));
#20612=CARTESIAN_POINT('',(0.,1.7,1.75));
#20613=CARTESIAN_POINT('',(1.97,1.7,1.75));
#20614=CARTESIAN_POINT('',(0.,1.7,1.75));
#20615=CARTESIAN_POINT('',(1.97,1.7,0.43));
#20616=CARTESIAN_POINT('',(1.97,1.7,0.43));
#20617=CARTESIAN_POINT('',(-1.97,1.7,0.43));
#20618=CARTESIAN_POINT('',(0.,1.7,0.43));
#20619=CARTESIAN_POINT('',(-1.97,1.7,1.75));
#20620=CARTESIAN_POINT('',(-1.97,1.7,0.43));
#20621=CARTESIAN_POINT('',(0.,1.7,1.75));
#20622=CARTESIAN_POINT('Origin',(-1.97,0.,1.415));
#20623=CARTESIAN_POINT('',(-1.97,-2.35,1.75));
#20624=CARTESIAN_POINT('',(-1.97,-2.35,1.75));
#20625=CARTESIAN_POINT('',(-1.97,-2.35,2.4));
#20626=CARTESIAN_POINT('',(-1.97,-2.35,2.4));
#20627=CARTESIAN_POINT('',(-1.97,2.35,2.4));
#20628=CARTESIAN_POINT('',(-1.97,2.35,2.4));
#20629=CARTESIAN_POINT('',(-1.97,2.35,1.75));
#20630=CARTESIAN_POINT('',(-1.97,2.35,1.75));
#20631=CARTESIAN_POINT('',(-1.97,1.7,1.75));
#20632=CARTESIAN_POINT('',(-1.97,0.78,0.43));
#20633=CARTESIAN_POINT('',(-1.97,0.78,0.43));
#20634=CARTESIAN_POINT('',(-1.97,0.78,1.55));
#20635=CARTESIAN_POINT('',(-1.97,0.78,1.55));
#20636=CARTESIAN_POINT('',(-1.97,-0.78,1.55));
#20637=CARTESIAN_POINT('',(-1.97,-0.78,1.55));
#20638=CARTESIAN_POINT('',(-1.97,-0.78,0.43));
#20639=CARTESIAN_POINT('',(-1.97,-0.78,0.43));
#20640=CARTESIAN_POINT('',(-1.97,-1.7,0.43));
#20641=CARTESIAN_POINT('Origin',(0.,-2.35,1.75));
#20642=CARTESIAN_POINT('',(1.97,-2.35,1.75));
#20643=CARTESIAN_POINT('',(1.97,-2.35,1.75));
#20644=CARTESIAN_POINT('',(0.,-2.35,1.75));
#20645=CARTESIAN_POINT('Origin',(0.,-2.35,2.4));
#20646=CARTESIAN_POINT('',(1.97,-2.35,2.4));
#20647=CARTESIAN_POINT('',(1.97,-2.35,2.4));
#20648=CARTESIAN_POINT('',(0.,-2.35,2.4));
#20649=CARTESIAN_POINT('Origin',(0.,2.35,2.4));
#20650=CARTESIAN_POINT('',(1.97,2.35,2.4));
#20651=CARTESIAN_POINT('',(1.97,2.35,2.4));
#20652=CARTESIAN_POINT('',(0.,2.35,2.4));
#20653=CARTESIAN_POINT('Origin',(0.,2.35,1.75));
#20654=CARTESIAN_POINT('',(1.97,2.35,1.75));
#20655=CARTESIAN_POINT('',(1.97,2.35,1.75));
#20656=CARTESIAN_POINT('',(0.,2.35,1.75));
#20657=CARTESIAN_POINT('Origin',(0.,1.7,1.75));
#20658=CARTESIAN_POINT('',(1.97,1.7,1.75));
#20659=CARTESIAN_POINT('Origin',(0.,0.78,0.43));
#20660=CARTESIAN_POINT('',(1.97,0.78,0.43));
#20661=CARTESIAN_POINT('',(1.97,0.78,0.43));
#20662=CARTESIAN_POINT('',(0.,0.78,0.43));
#20663=CARTESIAN_POINT('Origin',(0.,0.78,1.55));
#20664=CARTESIAN_POINT('',(1.97,0.78,1.55));
#20665=CARTESIAN_POINT('',(1.97,0.78,1.55));
#20666=CARTESIAN_POINT('',(0.,0.78,1.55));
#20667=CARTESIAN_POINT('Origin',(0.,-0.78,1.55));
#20668=CARTESIAN_POINT('',(1.97,-0.78,1.55));
#20669=CARTESIAN_POINT('',(1.97,-0.78,1.55));
#20670=CARTESIAN_POINT('',(0.,-0.78,1.55));
#20671=CARTESIAN_POINT('Origin',(0.,-0.78,0.43));
#20672=CARTESIAN_POINT('',(1.97,-0.78,0.43));
#20673=CARTESIAN_POINT('',(1.97,-0.78,0.43));
#20674=CARTESIAN_POINT('',(0.,-0.78,0.43));
#20675=CARTESIAN_POINT('Origin',(0.,-1.7,0.43));
#20676=CARTESIAN_POINT('',(1.97,-1.7,0.43));
#20677=CARTESIAN_POINT('Origin',(1.97,0.,1.415));
#23490=UNCERTAINTY_MEASURE_WITH_UNIT(LENGTH_MEASURE(0.001),#23588,
'DISTANCE_ACCURACY_VALUE',
'Maximum model space distance between geometric entities at asserted c
onnectivities');
#23522=UNCERTAINTY_MEASURE_WITH_UNIT(LENGTH_MEASURE(0.001),#23588,
'DISTANCE_ACCURACY_VALUE',
'Maximum model space distance between geometric entities at asserted c
onnectivities');
#23555=(
GEOMETRIC_REPRESENTATION_CONTEXT(3)
GLOBAL_UNCERTAINTY_ASSIGNED_CONTEXT((#23490))
GLOBAL_UNIT_ASSIGNED_CONTEXT((#23588,#23590,#23591))
REPRESENTATION_CONTEXT('','3D')
);
#23587=(
GEOMETRIC_REPRESENTATION_CONTEXT(3)
GLOBAL_UNCERTAINTY_ASSIGNED_CONTEXT((#23522))
GLOBAL_UNIT_ASSIGNED_CONTEXT((#23588,#23590,#23591))
REPRESENTATION_CONTEXT('','3D')
);
#23588=(
LENGTH_UNIT()
NAMED_UNIT(*)
SI_UNIT(.CENTI.,.METRE.)
);
#23590=(
NAMED_UNIT(*)
PLANE_ANGLE_UNIT()
SI_UNIT($,.RADIAN.)
);
#23591=(
NAMED_UNIT(*)
SI_UNIT($,.STERADIAN.)
SOLID_ANGLE_UNIT()
);
#23624=SHAPE_DEFINITION_REPRESENTATION(#23693,#23857);
#23693=PRODUCT_DEFINITION_SHAPE('',$,#23922);
#23857=SHAPE_REPRESENTATION('',(#13565),#23555);
#23889=PRODUCT_DEFINITION_CONTEXT('part definition',#24083,'design');
#23922=PRODUCT_DEFINITION('Block','Block',#23986,#23889);
#23986=PRODUCT_DEFINITION_FORMATION('',$,#24117);
#24083=APPLICATION_CONTEXT(
'Core Data for Automotive Mechanical Design Process');
#24084=PRODUCT_CONTEXT('part definition',#24083,'mechanical');
#24117=PRODUCT('Block','Block','Block',(#24084));
#24184=COLOUR_RGB('Dark Blue',0.08,0.2,0.34);
#24185=FILL_AREA_STYLE_COLOUR('',#24184);
#24186=FILL_AREA_STYLE('',(#24185));
#24187=SURFACE_STYLE_FILL_AREA(#24186);
#24188=SURFACE_SIDE_STYLE('',(#24187));
#24189=SURFACE_STYLE_USAGE(.BOTH.,#24188);
#24190=PRESENTATION_STYLE_ASSIGNMENT((#24189));
ENDSEC;
END-ISO-10303-21;
